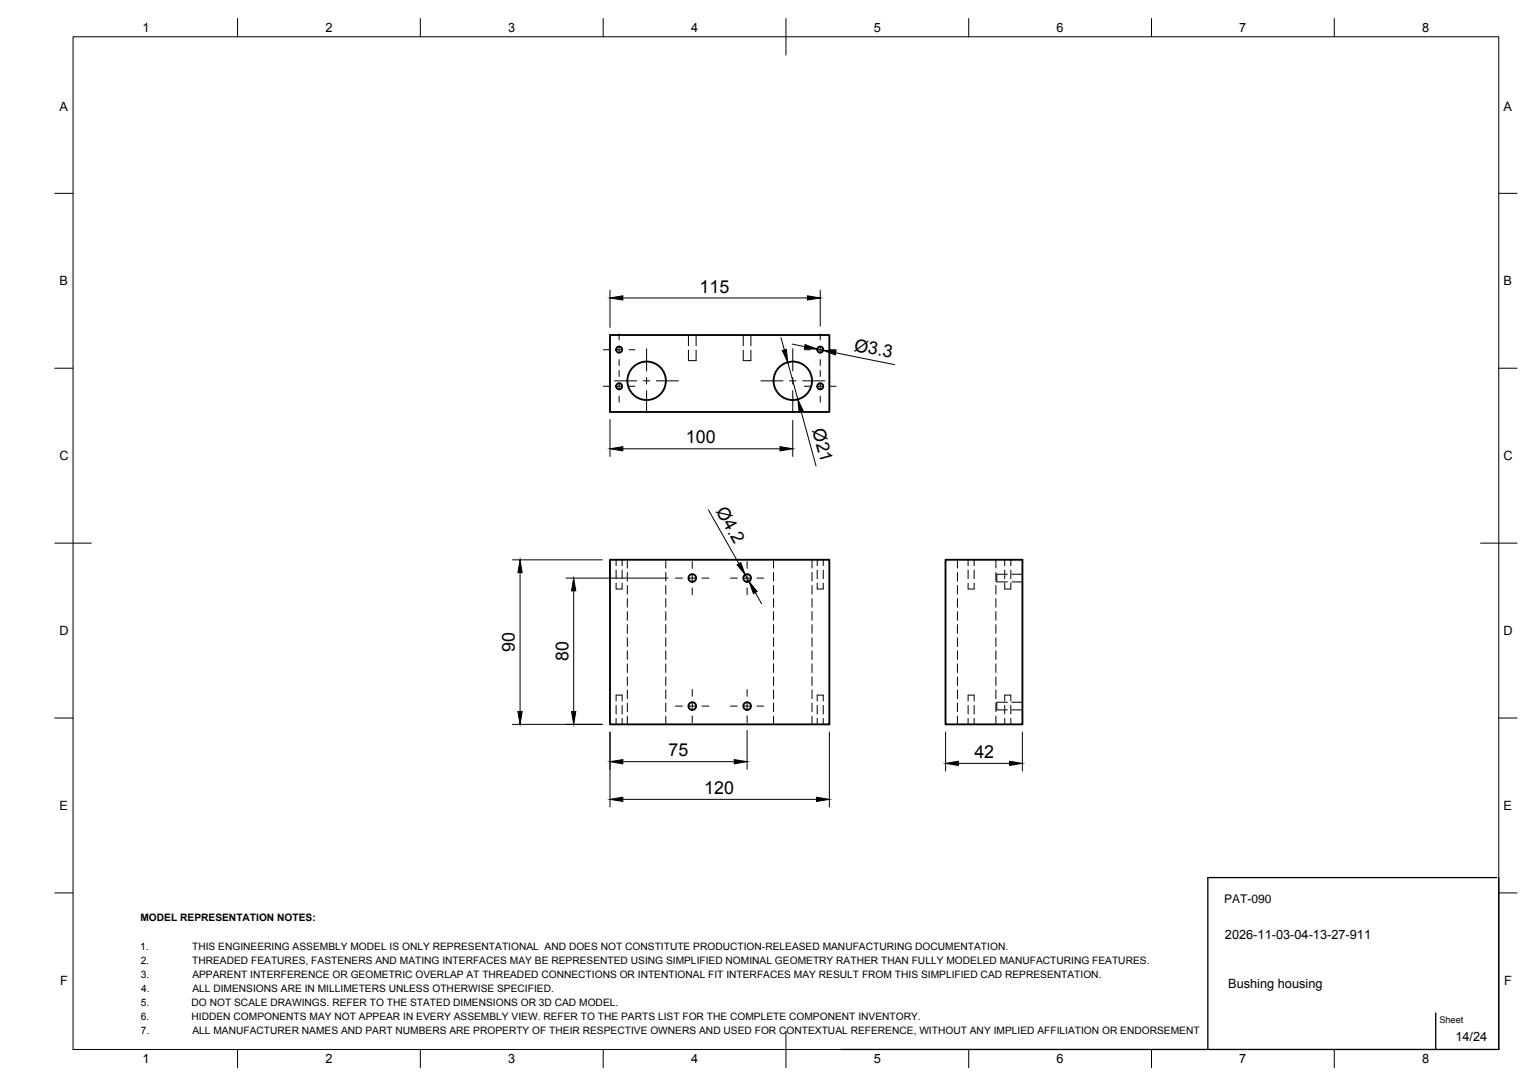
ISO-10303-21;
HEADER;
/* Generated by software containing ST-Developer
 * from STEP Tools, Inc. (www.steptools.com) 
 */

FILE_DESCRIPTION(
/* description */ ('Round-Shaft Linear Stage with Ball Bushings'),
/* implementation_level */ '2;1');

FILE_NAME(
/* name */ 'Bushing housing.step',
/* time_stamp */ '2026-10-27T10:47:55-07:00',
/* author */ (''),
/* organization */ (''),
/* preprocessor_version */ 'ST-DEVELOPER v20.2',
/* originating_system */ 'Autodesk Translation Framework v15.17.0.0',
/* authorisation */ '');

FILE_SCHEMA (('AUTOMOTIVE_DESIGN { 1 0 10303 214 3 1 1 }'));
ENDSEC;

DATA;
#10=MECHANICAL_DESIGN_GEOMETRIC_PRESENTATION_REPRESENTATION('',(#310),#7835);
#268=SHAPE_REPRESENTATION_RELATIONSHIP('SRR','None',#7957,#289);
#289=ADVANCED_BREP_SHAPE_REPRESENTATION('',(#330),#7821);
#310=STYLED_ITEM('',(#8123),#330);
#330=MANIFOLD_SOLID_BREP('Body1',#4401);
#387=FACE_BOUND('',#1046,.T.);
#388=FACE_BOUND('',#1047,.T.);
#389=FACE_BOUND('',#1048,.T.);
#390=FACE_BOUND('',#1049,.T.);
#391=FACE_BOUND('',#1050,.T.);
#392=FACE_BOUND('',#1051,.T.);
#393=FACE_BOUND('',#1054,.T.);
#394=FACE_BOUND('',#1055,.T.);
#395=FACE_BOUND('',#1056,.T.);
#396=FACE_BOUND('',#1057,.T.);
#397=FACE_BOUND('',#1058,.T.);
#398=FACE_BOUND('',#1059,.T.);
#399=FACE_BOUND('',#1061,.T.);
#400=FACE_BOUND('',#1062,.T.);
#401=FACE_BOUND('',#1063,.T.);
#402=FACE_BOUND('',#1064,.T.);
#522=PLANE('',#4827);
#523=PLANE('',#4831);
#524=PLANE('',#4835);
#525=PLANE('',#4839);
#526=PLANE('',#4843);
#527=PLANE('',#4847);
#528=PLANE('',#4851);
#529=PLANE('',#4855);
#530=PLANE('',#4859);
#531=PLANE('',#4863);
#532=PLANE('',#4867);
#533=PLANE('',#4871);
#534=PLANE('',#4878);
#535=PLANE('',#4879);
#536=PLANE('',#4880);
#537=PLANE('',#4881);
#538=PLANE('',#4882);
#539=PLANE('',#4883);
#714=FACE_OUTER_BOUND('',#1018,.T.);
#715=FACE_OUTER_BOUND('',#1019,.T.);
#716=FACE_OUTER_BOUND('',#1020,.T.);
#717=FACE_OUTER_BOUND('',#1021,.T.);
#718=FACE_OUTER_BOUND('',#1022,.T.);
#719=FACE_OUTER_BOUND('',#1023,.T.);
#720=FACE_OUTER_BOUND('',#1024,.T.);
#721=FACE_OUTER_BOUND('',#1025,.T.);
#722=FACE_OUTER_BOUND('',#1026,.T.);
#723=FACE_OUTER_BOUND('',#1027,.T.);
#724=FACE_OUTER_BOUND('',#1028,.T.);
#725=FACE_OUTER_BOUND('',#1029,.T.);
#726=FACE_OUTER_BOUND('',#1030,.T.);
#727=FACE_OUTER_BOUND('',#1031,.T.);
#728=FACE_OUTER_BOUND('',#1032,.T.);
#729=FACE_OUTER_BOUND('',#1033,.T.);
#730=FACE_OUTER_BOUND('',#1034,.T.);
#731=FACE_OUTER_BOUND('',#1035,.T.);
#732=FACE_OUTER_BOUND('',#1036,.T.);
#733=FACE_OUTER_BOUND('',#1037,.T.);
#734=FACE_OUTER_BOUND('',#1038,.T.);
#735=FACE_OUTER_BOUND('',#1039,.T.);
#736=FACE_OUTER_BOUND('',#1040,.T.);
#737=FACE_OUTER_BOUND('',#1041,.T.);
#738=FACE_OUTER_BOUND('',#1042,.T.);
#739=FACE_OUTER_BOUND('',#1043,.T.);
#740=FACE_OUTER_BOUND('',#1044,.T.);
#741=FACE_OUTER_BOUND('',#1045,.T.);
#742=FACE_OUTER_BOUND('',#1052,.T.);
#743=FACE_OUTER_BOUND('',#1053,.T.);
#744=FACE_OUTER_BOUND('',#1060,.T.);
#745=FACE_OUTER_BOUND('',#1065,.T.);
#1018=EDGE_LOOP('',(#3434,#3435,#3436,#3437));
#1019=EDGE_LOOP('',(#3438));
#1020=EDGE_LOOP('',(#3439,#3440,#3441,#3442));
#1021=EDGE_LOOP('',(#3443));
#1022=EDGE_LOOP('',(#3444,#3445,#3446,#3447));
#1023=EDGE_LOOP('',(#3448));
#1024=EDGE_LOOP('',(#3449,#3450,#3451,#3452));
#1025=EDGE_LOOP('',(#3453));
#1026=EDGE_LOOP('',(#3454,#3455,#3456,#3457));
#1027=EDGE_LOOP('',(#3458));
#1028=EDGE_LOOP('',(#3459,#3460,#3461,#3462));
#1029=EDGE_LOOP('',(#3463));
#1030=EDGE_LOOP('',(#3464,#3465,#3466,#3467));
#1031=EDGE_LOOP('',(#3468));
#1032=EDGE_LOOP('',(#3469,#3470,#3471,#3472));
#1033=EDGE_LOOP('',(#3473));
#1034=EDGE_LOOP('',(#3474,#3475,#3476,#3477));
#1035=EDGE_LOOP('',(#3478));
#1036=EDGE_LOOP('',(#3479,#3480,#3481,#3482));
#1037=EDGE_LOOP('',(#3483));
#1038=EDGE_LOOP('',(#3484,#3485,#3486,#3487));
#1039=EDGE_LOOP('',(#3488));
#1040=EDGE_LOOP('',(#3489,#3490,#3491,#3492));
#1041=EDGE_LOOP('',(#3493));
#1042=EDGE_LOOP('',(#3494,#3495,#3496,#3497));
#1043=EDGE_LOOP('',(#3498,#3499,#3500,#3501));
#1044=EDGE_LOOP('',(#3502,#3503,#3504,#3505));
#1045=EDGE_LOOP('',(#3506,#3507,#3508,#3509));
#1046=EDGE_LOOP('',(#3510));
#1047=EDGE_LOOP('',(#3511));
#1048=EDGE_LOOP('',(#3512));
#1049=EDGE_LOOP('',(#3513));
#1050=EDGE_LOOP('',(#3514));
#1051=EDGE_LOOP('',(#3515));
#1052=EDGE_LOOP('',(#3516,#3517,#3518,#3519));
#1053=EDGE_LOOP('',(#3520,#3521,#3522,#3523));
#1054=EDGE_LOOP('',(#3524));
#1055=EDGE_LOOP('',(#3525));
#1056=EDGE_LOOP('',(#3526));
#1057=EDGE_LOOP('',(#3527));
#1058=EDGE_LOOP('',(#3528));
#1059=EDGE_LOOP('',(#3529));
#1060=EDGE_LOOP('',(#3530,#3531,#3532,#3533));
#1061=EDGE_LOOP('',(#3534));
#1062=EDGE_LOOP('',(#3535));
#1063=EDGE_LOOP('',(#3536));
#1064=EDGE_LOOP('',(#3537));
#1065=EDGE_LOOP('',(#3538,#3539,#3540,#3541));
#1404=LINE('',#7049,#1744);
#1405=LINE('',#7056,#1745);
#1406=LINE('',#7063,#1746);
#1407=LINE('',#7070,#1747);
#1408=LINE('',#7077,#1748);
#1409=LINE('',#7084,#1749);
#1410=LINE('',#7091,#1750);
#1411=LINE('',#7098,#1751);
#1412=LINE('',#7105,#1752);
#1413=LINE('',#7112,#1753);
#1414=LINE('',#7119,#1754);
#1415=LINE('',#7126,#1755);
#1416=LINE('',#7133,#1756);
#1417=LINE('',#7139,#1757);
#1418=LINE('',#7144,#1758);
#1419=LINE('',#7146,#1759);
#1420=LINE('',#7148,#1760);
#1421=LINE('',#7149,#1761);
#1422=LINE('',#7152,#1762);
#1423=LINE('',#7154,#1763);
#1424=LINE('',#7155,#1764);
#1425=LINE('',#7158,#1765);
#1426=LINE('',#7160,#1766);
#1427=LINE('',#7161,#1767);
#1428=LINE('',#7163,#1768);
#1429=LINE('',#7164,#1769);
#1744=VECTOR('',#5685,0.165);
#1745=VECTOR('',#5694,0.165);
#1746=VECTOR('',#5703,0.165);
#1747=VECTOR('',#5712,0.165);
#1748=VECTOR('',#5721,0.165);
#1749=VECTOR('',#5730,0.165);
#1750=VECTOR('',#5739,0.165);
#1751=VECTOR('',#5748,0.165);
#1752=VECTOR('',#5757,0.210000000000001);
#1753=VECTOR('',#5766,0.210000000000001);
#1754=VECTOR('',#5775,0.210000000000001);
#1755=VECTOR('',#5784,0.210000000000001);
#1756=VECTOR('',#5793,1.05);
#1757=VECTOR('',#5800,1.05);
#1758=VECTOR('',#5805,1.);
#1759=VECTOR('',#5806,1.);
#1760=VECTOR('',#5807,1.);
#1761=VECTOR('',#5808,1.);
#1762=VECTOR('',#5811,1.);
#1763=VECTOR('',#5812,1.);
#1764=VECTOR('',#5813,1.);
#1765=VECTOR('',#5816,1.);
#1766=VECTOR('',#5817,1.);
#1767=VECTOR('',#5818,1.);
#1768=VECTOR('',#5821,1.);
#1769=VECTOR('',#5822,1.);
#1994=CIRCLE('',#4825,0.165);
#1995=CIRCLE('',#4826,0.165);
#1996=CIRCLE('',#4829,0.165);
#1997=CIRCLE('',#4830,0.165);
#1998=CIRCLE('',#4833,0.165);
#1999=CIRCLE('',#4834,0.165);
#2000=CIRCLE('',#4837,0.165);
#2001=CIRCLE('',#4838,0.165);
#2002=CIRCLE('',#4841,0.165);
#2003=CIRCLE('',#4842,0.165);
#2004=CIRCLE('',#4845,0.165);
#2005=CIRCLE('',#4846,0.165);
#2006=CIRCLE('',#4849,0.165);
#2007=CIRCLE('',#4850,0.165);
#2008=CIRCLE('',#4853,0.165);
#2009=CIRCLE('',#4854,0.165);
#2010=CIRCLE('',#4857,0.210000000000001);
#2011=CIRCLE('',#4858,0.210000000000001);
#2012=CIRCLE('',#4861,0.210000000000001);
#2013=CIRCLE('',#4862,0.210000000000001);
#2014=CIRCLE('',#4865,0.210000000000001);
#2015=CIRCLE('',#4866,0.210000000000001);
#2016=CIRCLE('',#4869,0.210000000000001);
#2017=CIRCLE('',#4870,0.210000000000001);
#2018=CIRCLE('',#4873,1.05);
#2019=CIRCLE('',#4874,1.05);
#2020=CIRCLE('',#4876,1.05);
#2021=CIRCLE('',#4877,1.05);
#2263=VERTEX_POINT('',#7046);
#2264=VERTEX_POINT('',#7048);
#2265=VERTEX_POINT('',#7053);
#2266=VERTEX_POINT('',#7055);
#2267=VERTEX_POINT('',#7060);
#2268=VERTEX_POINT('',#7062);
#2269=VERTEX_POINT('',#7067);
#2270=VERTEX_POINT('',#7069);
#2271=VERTEX_POINT('',#7074);
#2272=VERTEX_POINT('',#7076);
#2273=VERTEX_POINT('',#7081);
#2274=VERTEX_POINT('',#7083);
#2275=VERTEX_POINT('',#7088);
#2276=VERTEX_POINT('',#7090);
#2277=VERTEX_POINT('',#7095);
#2278=VERTEX_POINT('',#7097);
#2279=VERTEX_POINT('',#7102);
#2280=VERTEX_POINT('',#7104);
#2281=VERTEX_POINT('',#7109);
#2282=VERTEX_POINT('',#7111);
#2283=VERTEX_POINT('',#7116);
#2284=VERTEX_POINT('',#7118);
#2285=VERTEX_POINT('',#7123);
#2286=VERTEX_POINT('',#7125);
#2287=VERTEX_POINT('',#7130);
#2288=VERTEX_POINT('',#7132);
#2289=VERTEX_POINT('',#7136);
#2290=VERTEX_POINT('',#7138);
#2291=VERTEX_POINT('',#7142);
#2292=VERTEX_POINT('',#7143);
#2293=VERTEX_POINT('',#7145);
#2294=VERTEX_POINT('',#7147);
#2295=VERTEX_POINT('',#7151);
#2296=VERTEX_POINT('',#7153);
#2297=VERTEX_POINT('',#7157);
#2298=VERTEX_POINT('',#7159);
#2685=EDGE_CURVE('',#2263,#2263,#1994,.T.);
#2686=EDGE_CURVE('',#2263,#2264,#1404,.T.);
#2687=EDGE_CURVE('',#2264,#2264,#1995,.T.);
#2688=EDGE_CURVE('',#2265,#2265,#1996,.T.);
#2689=EDGE_CURVE('',#2265,#2266,#1405,.T.);
#2690=EDGE_CURVE('',#2266,#2266,#1997,.T.);
#2691=EDGE_CURVE('',#2267,#2267,#1998,.T.);
#2692=EDGE_CURVE('',#2267,#2268,#1406,.T.);
#2693=EDGE_CURVE('',#2268,#2268,#1999,.T.);
#2694=EDGE_CURVE('',#2269,#2269,#2000,.T.);
#2695=EDGE_CURVE('',#2269,#2270,#1407,.T.);
#2696=EDGE_CURVE('',#2270,#2270,#2001,.T.);
#2697=EDGE_CURVE('',#2271,#2271,#2002,.T.);
#2698=EDGE_CURVE('',#2271,#2272,#1408,.T.);
#2699=EDGE_CURVE('',#2272,#2272,#2003,.T.);
#2700=EDGE_CURVE('',#2273,#2273,#2004,.T.);
#2701=EDGE_CURVE('',#2273,#2274,#1409,.T.);
#2702=EDGE_CURVE('',#2274,#2274,#2005,.T.);
#2703=EDGE_CURVE('',#2275,#2275,#2006,.T.);
#2704=EDGE_CURVE('',#2275,#2276,#1410,.T.);
#2705=EDGE_CURVE('',#2276,#2276,#2007,.T.);
#2706=EDGE_CURVE('',#2277,#2277,#2008,.T.);
#2707=EDGE_CURVE('',#2277,#2278,#1411,.T.);
#2708=EDGE_CURVE('',#2278,#2278,#2009,.T.);
#2709=EDGE_CURVE('',#2279,#2279,#2010,.T.);
#2710=EDGE_CURVE('',#2279,#2280,#1412,.T.);
#2711=EDGE_CURVE('',#2280,#2280,#2011,.T.);
#2712=EDGE_CURVE('',#2281,#2281,#2012,.T.);
#2713=EDGE_CURVE('',#2281,#2282,#1413,.T.);
#2714=EDGE_CURVE('',#2282,#2282,#2013,.T.);
#2715=EDGE_CURVE('',#2283,#2283,#2014,.T.);
#2716=EDGE_CURVE('',#2283,#2284,#1414,.T.);
#2717=EDGE_CURVE('',#2284,#2284,#2015,.T.);
#2718=EDGE_CURVE('',#2285,#2285,#2016,.T.);
#2719=EDGE_CURVE('',#2285,#2286,#1415,.T.);
#2720=EDGE_CURVE('',#2286,#2286,#2017,.T.);
#2721=EDGE_CURVE('',#2287,#2287,#2018,.T.);
#2722=EDGE_CURVE('',#2287,#2288,#1416,.T.);
#2723=EDGE_CURVE('',#2288,#2288,#2019,.T.);
#2724=EDGE_CURVE('',#2289,#2289,#2020,.T.);
#2725=EDGE_CURVE('',#2289,#2290,#1417,.T.);
#2726=EDGE_CURVE('',#2290,#2290,#2021,.T.);
#2727=EDGE_CURVE('',#2291,#2292,#1418,.T.);
#2728=EDGE_CURVE('',#2292,#2293,#1419,.T.);
#2729=EDGE_CURVE('',#2294,#2293,#1420,.T.);
#2730=EDGE_CURVE('',#2291,#2294,#1421,.T.);
#2731=EDGE_CURVE('',#2295,#2291,#1422,.T.);
#2732=EDGE_CURVE('',#2296,#2294,#1423,.T.);
#2733=EDGE_CURVE('',#2295,#2296,#1424,.T.);
#2734=EDGE_CURVE('',#2297,#2295,#1425,.T.);
#2735=EDGE_CURVE('',#2298,#2296,#1426,.T.);
#2736=EDGE_CURVE('',#2297,#2298,#1427,.T.);
#2737=EDGE_CURVE('',#2292,#2297,#1428,.T.);
#2738=EDGE_CURVE('',#2293,#2298,#1429,.T.);
#3434=ORIENTED_EDGE('',*,*,#2685,.F.);
#3435=ORIENTED_EDGE('',*,*,#2686,.T.);
#3436=ORIENTED_EDGE('',*,*,#2687,.F.);
#3437=ORIENTED_EDGE('',*,*,#2686,.F.);
#3438=ORIENTED_EDGE('',*,*,#2685,.T.);
#3439=ORIENTED_EDGE('',*,*,#2688,.F.);
#3440=ORIENTED_EDGE('',*,*,#2689,.T.);
#3441=ORIENTED_EDGE('',*,*,#2690,.F.);
#3442=ORIENTED_EDGE('',*,*,#2689,.F.);
#3443=ORIENTED_EDGE('',*,*,#2688,.T.);
#3444=ORIENTED_EDGE('',*,*,#2691,.F.);
#3445=ORIENTED_EDGE('',*,*,#2692,.T.);
#3446=ORIENTED_EDGE('',*,*,#2693,.F.);
#3447=ORIENTED_EDGE('',*,*,#2692,.F.);
#3448=ORIENTED_EDGE('',*,*,#2691,.T.);
#3449=ORIENTED_EDGE('',*,*,#2694,.F.);
#3450=ORIENTED_EDGE('',*,*,#2695,.T.);
#3451=ORIENTED_EDGE('',*,*,#2696,.F.);
#3452=ORIENTED_EDGE('',*,*,#2695,.F.);
#3453=ORIENTED_EDGE('',*,*,#2694,.T.);
#3454=ORIENTED_EDGE('',*,*,#2697,.F.);
#3455=ORIENTED_EDGE('',*,*,#2698,.T.);
#3456=ORIENTED_EDGE('',*,*,#2699,.T.);
#3457=ORIENTED_EDGE('',*,*,#2698,.F.);
#3458=ORIENTED_EDGE('',*,*,#2699,.F.);
#3459=ORIENTED_EDGE('',*,*,#2700,.F.);
#3460=ORIENTED_EDGE('',*,*,#2701,.T.);
#3461=ORIENTED_EDGE('',*,*,#2702,.T.);
#3462=ORIENTED_EDGE('',*,*,#2701,.F.);
#3463=ORIENTED_EDGE('',*,*,#2702,.F.);
#3464=ORIENTED_EDGE('',*,*,#2703,.F.);
#3465=ORIENTED_EDGE('',*,*,#2704,.T.);
#3466=ORIENTED_EDGE('',*,*,#2705,.T.);
#3467=ORIENTED_EDGE('',*,*,#2704,.F.);
#3468=ORIENTED_EDGE('',*,*,#2705,.F.);
#3469=ORIENTED_EDGE('',*,*,#2706,.F.);
#3470=ORIENTED_EDGE('',*,*,#2707,.T.);
#3471=ORIENTED_EDGE('',*,*,#2708,.T.);
#3472=ORIENTED_EDGE('',*,*,#2707,.F.);
#3473=ORIENTED_EDGE('',*,*,#2708,.F.);
#3474=ORIENTED_EDGE('',*,*,#2709,.F.);
#3475=ORIENTED_EDGE('',*,*,#2710,.T.);
#3476=ORIENTED_EDGE('',*,*,#2711,.F.);
#3477=ORIENTED_EDGE('',*,*,#2710,.F.);
#3478=ORIENTED_EDGE('',*,*,#2709,.T.);
#3479=ORIENTED_EDGE('',*,*,#2712,.F.);
#3480=ORIENTED_EDGE('',*,*,#2713,.T.);
#3481=ORIENTED_EDGE('',*,*,#2714,.F.);
#3482=ORIENTED_EDGE('',*,*,#2713,.F.);
#3483=ORIENTED_EDGE('',*,*,#2712,.T.);
#3484=ORIENTED_EDGE('',*,*,#2715,.F.);
#3485=ORIENTED_EDGE('',*,*,#2716,.T.);
#3486=ORIENTED_EDGE('',*,*,#2717,.F.);
#3487=ORIENTED_EDGE('',*,*,#2716,.F.);
#3488=ORIENTED_EDGE('',*,*,#2715,.T.);
#3489=ORIENTED_EDGE('',*,*,#2718,.F.);
#3490=ORIENTED_EDGE('',*,*,#2719,.T.);
#3491=ORIENTED_EDGE('',*,*,#2720,.F.);
#3492=ORIENTED_EDGE('',*,*,#2719,.F.);
#3493=ORIENTED_EDGE('',*,*,#2718,.T.);
#3494=ORIENTED_EDGE('',*,*,#2721,.F.);
#3495=ORIENTED_EDGE('',*,*,#2722,.T.);
#3496=ORIENTED_EDGE('',*,*,#2723,.F.);
#3497=ORIENTED_EDGE('',*,*,#2722,.F.);
#3498=ORIENTED_EDGE('',*,*,#2724,.F.);
#3499=ORIENTED_EDGE('',*,*,#2725,.T.);
#3500=ORIENTED_EDGE('',*,*,#2726,.F.);
#3501=ORIENTED_EDGE('',*,*,#2725,.F.);
#3502=ORIENTED_EDGE('',*,*,#2727,.T.);
#3503=ORIENTED_EDGE('',*,*,#2728,.T.);
#3504=ORIENTED_EDGE('',*,*,#2729,.F.);
#3505=ORIENTED_EDGE('',*,*,#2730,.F.);
#3506=ORIENTED_EDGE('',*,*,#2731,.T.);
#3507=ORIENTED_EDGE('',*,*,#2730,.T.);
#3508=ORIENTED_EDGE('',*,*,#2732,.F.);
#3509=ORIENTED_EDGE('',*,*,#2733,.F.);
#3510=ORIENTED_EDGE('',*,*,#2726,.T.);
#3511=ORIENTED_EDGE('',*,*,#2723,.T.);
#3512=ORIENTED_EDGE('',*,*,#2696,.T.);
#3513=ORIENTED_EDGE('',*,*,#2693,.T.);
#3514=ORIENTED_EDGE('',*,*,#2690,.T.);
#3515=ORIENTED_EDGE('',*,*,#2687,.T.);
#3516=ORIENTED_EDGE('',*,*,#2734,.T.);
#3517=ORIENTED_EDGE('',*,*,#2733,.T.);
#3518=ORIENTED_EDGE('',*,*,#2735,.F.);
#3519=ORIENTED_EDGE('',*,*,#2736,.F.);
#3520=ORIENTED_EDGE('',*,*,#2737,.T.);
#3521=ORIENTED_EDGE('',*,*,#2736,.T.);
#3522=ORIENTED_EDGE('',*,*,#2738,.F.);
#3523=ORIENTED_EDGE('',*,*,#2728,.F.);
#3524=ORIENTED_EDGE('',*,*,#2724,.T.);
#3525=ORIENTED_EDGE('',*,*,#2721,.T.);
#3526=ORIENTED_EDGE('',*,*,#2706,.T.);
#3527=ORIENTED_EDGE('',*,*,#2703,.T.);
#3528=ORIENTED_EDGE('',*,*,#2700,.T.);
#3529=ORIENTED_EDGE('',*,*,#2697,.T.);
#3530=ORIENTED_EDGE('',*,*,#2738,.T.);
#3531=ORIENTED_EDGE('',*,*,#2735,.T.);
#3532=ORIENTED_EDGE('',*,*,#2732,.T.);
#3533=ORIENTED_EDGE('',*,*,#2729,.T.);
#3534=ORIENTED_EDGE('',*,*,#2711,.T.);
#3535=ORIENTED_EDGE('',*,*,#2714,.T.);
#3536=ORIENTED_EDGE('',*,*,#2717,.T.);
#3537=ORIENTED_EDGE('',*,*,#2720,.T.);
#3538=ORIENTED_EDGE('',*,*,#2737,.F.);
#3539=ORIENTED_EDGE('',*,*,#2727,.F.);
#3540=ORIENTED_EDGE('',*,*,#2731,.F.);
#3541=ORIENTED_EDGE('',*,*,#2734,.F.);
#4082=CYLINDRICAL_SURFACE('',#4824,0.165);
#4083=CYLINDRICAL_SURFACE('',#4828,0.165);
#4084=CYLINDRICAL_SURFACE('',#4832,0.165);
#4085=CYLINDRICAL_SURFACE('',#4836,0.165);
#4086=CYLINDRICAL_SURFACE('',#4840,0.165);
#4087=CYLINDRICAL_SURFACE('',#4844,0.165);
#4088=CYLINDRICAL_SURFACE('',#4848,0.165);
#4089=CYLINDRICAL_SURFACE('',#4852,0.165);
#4090=CYLINDRICAL_SURFACE('',#4856,0.210000000000001);
#4091=CYLINDRICAL_SURFACE('',#4860,0.210000000000001);
#4092=CYLINDRICAL_SURFACE('',#4864,0.210000000000001);
#4093=CYLINDRICAL_SURFACE('',#4868,0.210000000000001);
#4094=CYLINDRICAL_SURFACE('',#4872,1.05);
#4095=CYLINDRICAL_SURFACE('',#4875,1.05);
#4233=ADVANCED_FACE('',(#714),#4082,.F.);
#4234=ADVANCED_FACE('',(#715),#522,.T.);
#4235=ADVANCED_FACE('',(#716),#4083,.F.);
#4236=ADVANCED_FACE('',(#717),#523,.T.);
#4237=ADVANCED_FACE('',(#718),#4084,.F.);
#4238=ADVANCED_FACE('',(#719),#524,.T.);
#4239=ADVANCED_FACE('',(#720),#4085,.F.);
#4240=ADVANCED_FACE('',(#721),#525,.T.);
#4241=ADVANCED_FACE('',(#722),#4086,.F.);
#4242=ADVANCED_FACE('',(#723),#526,.F.);
#4243=ADVANCED_FACE('',(#724),#4087,.F.);
#4244=ADVANCED_FACE('',(#725),#527,.F.);
#4245=ADVANCED_FACE('',(#726),#4088,.F.);
#4246=ADVANCED_FACE('',(#727),#528,.F.);
#4247=ADVANCED_FACE('',(#728),#4089,.F.);
#4248=ADVANCED_FACE('',(#729),#529,.F.);
#4249=ADVANCED_FACE('',(#730),#4090,.F.);
#4250=ADVANCED_FACE('',(#731),#530,.T.);
#4251=ADVANCED_FACE('',(#732),#4091,.F.);
#4252=ADVANCED_FACE('',(#733),#531,.T.);
#4253=ADVANCED_FACE('',(#734),#4092,.F.);
#4254=ADVANCED_FACE('',(#735),#532,.T.);
#4255=ADVANCED_FACE('',(#736),#4093,.F.);
#4256=ADVANCED_FACE('',(#737),#533,.T.);
#4257=ADVANCED_FACE('',(#738),#4094,.F.);
#4258=ADVANCED_FACE('',(#739),#4095,.F.);
#4259=ADVANCED_FACE('',(#740),#534,.T.);
#4260=ADVANCED_FACE('',(#741,#387,#388,#389,#390,#391,#392),#535,.T.);
#4261=ADVANCED_FACE('',(#742),#536,.T.);
#4262=ADVANCED_FACE('',(#743,#393,#394,#395,#396,#397,#398),#537,.T.);
#4263=ADVANCED_FACE('',(#744,#399,#400,#401,#402),#538,.T.);
#4264=ADVANCED_FACE('',(#745),#539,.F.);
#4401=CLOSED_SHELL('',(#4233,#4234,#4235,#4236,#4237,#4238,#4239,#4240,
#4241,#4242,#4243,#4244,#4245,#4246,#4247,#4248,#4249,#4250,#4251,#4252,
#4253,#4254,#4255,#4256,#4257,#4258,#4259,#4260,#4261,#4262,#4263,#4264));
#4823=AXIS2_PLACEMENT_3D('',#7044,#5679,#5680);
#4824=AXIS2_PLACEMENT_3D('',#7045,#5681,#5682);
#4825=AXIS2_PLACEMENT_3D('',#7047,#5683,#5684);
#4826=AXIS2_PLACEMENT_3D('',#7050,#5686,#5687);
#4827=AXIS2_PLACEMENT_3D('',#7051,#5688,#5689);
#4828=AXIS2_PLACEMENT_3D('',#7052,#5690,#5691);
#4829=AXIS2_PLACEMENT_3D('',#7054,#5692,#5693);
#4830=AXIS2_PLACEMENT_3D('',#7057,#5695,#5696);
#4831=AXIS2_PLACEMENT_3D('',#7058,#5697,#5698);
#4832=AXIS2_PLACEMENT_3D('',#7059,#5699,#5700);
#4833=AXIS2_PLACEMENT_3D('',#7061,#5701,#5702);
#4834=AXIS2_PLACEMENT_3D('',#7064,#5704,#5705);
#4835=AXIS2_PLACEMENT_3D('',#7065,#5706,#5707);
#4836=AXIS2_PLACEMENT_3D('',#7066,#5708,#5709);
#4837=AXIS2_PLACEMENT_3D('',#7068,#5710,#5711);
#4838=AXIS2_PLACEMENT_3D('',#7071,#5713,#5714);
#4839=AXIS2_PLACEMENT_3D('',#7072,#5715,#5716);
#4840=AXIS2_PLACEMENT_3D('',#7073,#5717,#5718);
#4841=AXIS2_PLACEMENT_3D('',#7075,#5719,#5720);
#4842=AXIS2_PLACEMENT_3D('',#7078,#5722,#5723);
#4843=AXIS2_PLACEMENT_3D('',#7079,#5724,#5725);
#4844=AXIS2_PLACEMENT_3D('',#7080,#5726,#5727);
#4845=AXIS2_PLACEMENT_3D('',#7082,#5728,#5729);
#4846=AXIS2_PLACEMENT_3D('',#7085,#5731,#5732);
#4847=AXIS2_PLACEMENT_3D('',#7086,#5733,#5734);
#4848=AXIS2_PLACEMENT_3D('',#7087,#5735,#5736);
#4849=AXIS2_PLACEMENT_3D('',#7089,#5737,#5738);
#4850=AXIS2_PLACEMENT_3D('',#7092,#5740,#5741);
#4851=AXIS2_PLACEMENT_3D('',#7093,#5742,#5743);
#4852=AXIS2_PLACEMENT_3D('',#7094,#5744,#5745);
#4853=AXIS2_PLACEMENT_3D('',#7096,#5746,#5747);
#4854=AXIS2_PLACEMENT_3D('',#7099,#5749,#5750);
#4855=AXIS2_PLACEMENT_3D('',#7100,#5751,#5752);
#4856=AXIS2_PLACEMENT_3D('',#7101,#5753,#5754);
#4857=AXIS2_PLACEMENT_3D('',#7103,#5755,#5756);
#4858=AXIS2_PLACEMENT_3D('',#7106,#5758,#5759);
#4859=AXIS2_PLACEMENT_3D('',#7107,#5760,#5761);
#4860=AXIS2_PLACEMENT_3D('',#7108,#5762,#5763);
#4861=AXIS2_PLACEMENT_3D('',#7110,#5764,#5765);
#4862=AXIS2_PLACEMENT_3D('',#7113,#5767,#5768);
#4863=AXIS2_PLACEMENT_3D('',#7114,#5769,#5770);
#4864=AXIS2_PLACEMENT_3D('',#7115,#5771,#5772);
#4865=AXIS2_PLACEMENT_3D('',#7117,#5773,#5774);
#4866=AXIS2_PLACEMENT_3D('',#7120,#5776,#5777);
#4867=AXIS2_PLACEMENT_3D('',#7121,#5778,#5779);
#4868=AXIS2_PLACEMENT_3D('',#7122,#5780,#5781);
#4869=AXIS2_PLACEMENT_3D('',#7124,#5782,#5783);
#4870=AXIS2_PLACEMENT_3D('',#7127,#5785,#5786);
#4871=AXIS2_PLACEMENT_3D('',#7128,#5787,#5788);
#4872=AXIS2_PLACEMENT_3D('',#7129,#5789,#5790);
#4873=AXIS2_PLACEMENT_3D('',#7131,#5791,#5792);
#4874=AXIS2_PLACEMENT_3D('',#7134,#5794,#5795);
#4875=AXIS2_PLACEMENT_3D('',#7135,#5796,#5797);
#4876=AXIS2_PLACEMENT_3D('',#7137,#5798,#5799);
#4877=AXIS2_PLACEMENT_3D('',#7140,#5801,#5802);
#4878=AXIS2_PLACEMENT_3D('',#7141,#5803,#5804);
#4879=AXIS2_PLACEMENT_3D('',#7150,#5809,#5810);
#4880=AXIS2_PLACEMENT_3D('',#7156,#5814,#5815);
#4881=AXIS2_PLACEMENT_3D('',#7162,#5819,#5820);
#4882=AXIS2_PLACEMENT_3D('',#7165,#5823,#5824);
#4883=AXIS2_PLACEMENT_3D('',#7166,#5825,#5826);
#5679=DIRECTION('axis',(0.,0.,1.));
#5680=DIRECTION('refdir',(1.,0.,0.));
#5681=DIRECTION('center_axis',(1.,0.,0.));
#5682=DIRECTION('ref_axis',(0.,0.,-1.));
#5683=DIRECTION('center_axis',(1.,0.,0.));
#5684=DIRECTION('ref_axis',(0.,0.,-1.));
#5685=DIRECTION('',(1.,0.,0.));
#5686=DIRECTION('center_axis',(-1.,0.,0.));
#5687=DIRECTION('ref_axis',(0.,0.,-1.));
#5688=DIRECTION('center_axis',(1.,0.,0.));
#5689=DIRECTION('ref_axis',(0.,0.,-1.));
#5690=DIRECTION('center_axis',(1.,0.,0.));
#5691=DIRECTION('ref_axis',(0.,0.,-1.));
#5692=DIRECTION('center_axis',(1.,0.,0.));
#5693=DIRECTION('ref_axis',(0.,0.,-1.));
#5694=DIRECTION('',(1.,0.,0.));
#5695=DIRECTION('center_axis',(-1.,0.,0.));
#5696=DIRECTION('ref_axis',(0.,0.,-1.));
#5697=DIRECTION('center_axis',(1.,0.,0.));
#5698=DIRECTION('ref_axis',(0.,0.,-1.));
#5699=DIRECTION('center_axis',(1.,0.,0.));
#5700=DIRECTION('ref_axis',(0.,0.,-1.));
#5701=DIRECTION('center_axis',(1.,0.,0.));
#5702=DIRECTION('ref_axis',(0.,0.,-1.));
#5703=DIRECTION('',(1.,0.,0.));
#5704=DIRECTION('center_axis',(-1.,0.,0.));
#5705=DIRECTION('ref_axis',(0.,0.,-1.));
#5706=DIRECTION('center_axis',(1.,0.,0.));
#5707=DIRECTION('ref_axis',(0.,0.,-1.));
#5708=DIRECTION('center_axis',(1.,0.,0.));
#5709=DIRECTION('ref_axis',(0.,0.,-1.));
#5710=DIRECTION('center_axis',(1.,0.,0.));
#5711=DIRECTION('ref_axis',(0.,0.,-1.));
#5712=DIRECTION('',(1.,0.,0.));
#5713=DIRECTION('center_axis',(-1.,0.,0.));
#5714=DIRECTION('ref_axis',(0.,0.,-1.));
#5715=DIRECTION('center_axis',(1.,0.,0.));
#5716=DIRECTION('ref_axis',(0.,0.,-1.));
#5717=DIRECTION('center_axis',(1.,0.,0.));
#5718=DIRECTION('ref_axis',(0.,0.,-1.));
#5719=DIRECTION('center_axis',(1.,0.,0.));
#5720=DIRECTION('ref_axis',(0.,0.,-1.));
#5721=DIRECTION('',(1.,0.,0.));
#5722=DIRECTION('center_axis',(1.,0.,0.));
#5723=DIRECTION('ref_axis',(0.,0.,-1.));
#5724=DIRECTION('center_axis',(1.,0.,0.));
#5725=DIRECTION('ref_axis',(0.,0.,-1.));
#5726=DIRECTION('center_axis',(1.,0.,0.));
#5727=DIRECTION('ref_axis',(0.,0.,-1.));
#5728=DIRECTION('center_axis',(1.,0.,0.));
#5729=DIRECTION('ref_axis',(0.,0.,-1.));
#5730=DIRECTION('',(1.,0.,0.));
#5731=DIRECTION('center_axis',(1.,0.,0.));
#5732=DIRECTION('ref_axis',(0.,0.,-1.));
#5733=DIRECTION('center_axis',(1.,0.,0.));
#5734=DIRECTION('ref_axis',(0.,0.,-1.));
#5735=DIRECTION('center_axis',(1.,0.,0.));
#5736=DIRECTION('ref_axis',(0.,0.,-1.));
#5737=DIRECTION('center_axis',(1.,0.,0.));
#5738=DIRECTION('ref_axis',(0.,0.,-1.));
#5739=DIRECTION('',(1.,0.,0.));
#5740=DIRECTION('center_axis',(1.,0.,0.));
#5741=DIRECTION('ref_axis',(0.,0.,-1.));
#5742=DIRECTION('center_axis',(1.,0.,0.));
#5743=DIRECTION('ref_axis',(0.,0.,-1.));
#5744=DIRECTION('center_axis',(1.,0.,0.));
#5745=DIRECTION('ref_axis',(0.,0.,-1.));
#5746=DIRECTION('center_axis',(1.,0.,0.));
#5747=DIRECTION('ref_axis',(0.,0.,-1.));
#5748=DIRECTION('',(1.,0.,0.));
#5749=DIRECTION('center_axis',(1.,0.,0.));
#5750=DIRECTION('ref_axis',(0.,0.,-1.));
#5751=DIRECTION('center_axis',(1.,0.,0.));
#5752=DIRECTION('ref_axis',(0.,0.,-1.));
#5753=DIRECTION('center_axis',(0.,0.,1.));
#5754=DIRECTION('ref_axis',(1.,0.,0.));
#5755=DIRECTION('center_axis',(0.,0.,1.));
#5756=DIRECTION('ref_axis',(1.,0.,0.));
#5757=DIRECTION('',(0.,0.,1.));
#5758=DIRECTION('center_axis',(0.,0.,-1.));
#5759=DIRECTION('ref_axis',(1.,0.,0.));
#5760=DIRECTION('center_axis',(0.,0.,1.));
#5761=DIRECTION('ref_axis',(1.,0.,0.));
#5762=DIRECTION('center_axis',(0.,0.,1.));
#5763=DIRECTION('ref_axis',(1.,0.,0.));
#5764=DIRECTION('center_axis',(0.,0.,1.));
#5765=DIRECTION('ref_axis',(1.,0.,0.));
#5766=DIRECTION('',(0.,0.,1.));
#5767=DIRECTION('center_axis',(0.,0.,-1.));
#5768=DIRECTION('ref_axis',(1.,0.,0.));
#5769=DIRECTION('center_axis',(0.,0.,1.));
#5770=DIRECTION('ref_axis',(1.,0.,0.));
#5771=DIRECTION('center_axis',(0.,0.,1.));
#5772=DIRECTION('ref_axis',(1.,0.,0.));
#5773=DIRECTION('center_axis',(0.,0.,1.));
#5774=DIRECTION('ref_axis',(1.,0.,0.));
#5775=DIRECTION('',(0.,0.,1.));
#5776=DIRECTION('center_axis',(0.,0.,-1.));
#5777=DIRECTION('ref_axis',(1.,0.,0.));
#5778=DIRECTION('center_axis',(0.,0.,1.));
#5779=DIRECTION('ref_axis',(1.,0.,0.));
#5780=DIRECTION('center_axis',(0.,0.,1.));
#5781=DIRECTION('ref_axis',(1.,0.,0.));
#5782=DIRECTION('center_axis',(0.,0.,1.));
#5783=DIRECTION('ref_axis',(1.,0.,0.));
#5784=DIRECTION('',(0.,0.,1.));
#5785=DIRECTION('center_axis',(0.,0.,-1.));
#5786=DIRECTION('ref_axis',(1.,0.,0.));
#5787=DIRECTION('center_axis',(0.,0.,1.));
#5788=DIRECTION('ref_axis',(1.,0.,0.));
#5789=DIRECTION('center_axis',(1.,0.,0.));
#5790=DIRECTION('ref_axis',(0.,0.,-1.));
#5791=DIRECTION('center_axis',(1.,0.,0.));
#5792=DIRECTION('ref_axis',(0.,0.,-1.));
#5793=DIRECTION('',(1.,0.,0.));
#5794=DIRECTION('center_axis',(-1.,0.,0.));
#5795=DIRECTION('ref_axis',(0.,0.,-1.));
#5796=DIRECTION('center_axis',(1.,0.,0.));
#5797=DIRECTION('ref_axis',(0.,0.,-1.));
#5798=DIRECTION('center_axis',(1.,0.,0.));
#5799=DIRECTION('ref_axis',(0.,0.,-1.));
#5800=DIRECTION('',(1.,0.,0.));
#5801=DIRECTION('center_axis',(-1.,0.,0.));
#5802=DIRECTION('ref_axis',(0.,0.,-1.));
#5803=DIRECTION('center_axis',(0.,1.,0.));
#5804=DIRECTION('ref_axis',(-1.,0.,0.));
#5805=DIRECTION('',(-1.,0.,0.));
#5806=DIRECTION('',(0.,0.,1.));
#5807=DIRECTION('',(-1.,0.,0.));
#5808=DIRECTION('',(0.,0.,1.));
#5809=DIRECTION('center_axis',(1.,0.,0.));
#5810=DIRECTION('ref_axis',(0.,1.,0.));
#5811=DIRECTION('',(0.,1.,0.));
#5812=DIRECTION('',(0.,1.,0.));
#5813=DIRECTION('',(0.,0.,1.));
#5814=DIRECTION('center_axis',(0.,-1.,0.));
#5815=DIRECTION('ref_axis',(1.,0.,0.));
#5816=DIRECTION('',(1.,0.,0.));
#5817=DIRECTION('',(1.,0.,0.));
#5818=DIRECTION('',(0.,0.,1.));
#5819=DIRECTION('center_axis',(-1.,0.,0.));
#5820=DIRECTION('ref_axis',(0.,-1.,0.));
#5821=DIRECTION('',(0.,-1.,0.));
#5822=DIRECTION('',(0.,-1.,0.));
#5823=DIRECTION('center_axis',(0.,0.,1.));
#5824=DIRECTION('ref_axis',(1.,0.,0.));
#5825=DIRECTION('center_axis',(0.,0.,1.));
#5826=DIRECTION('ref_axis',(1.,0.,0.));
#7044=CARTESIAN_POINT('',(0.,0.,0.));
#7045=CARTESIAN_POINT('Origin',(17.9,5.5,3.));
#7046=CARTESIAN_POINT('',(17.9,5.5,3.165));
#7047=CARTESIAN_POINT('Origin',(17.9,5.5,3.));
#7048=CARTESIAN_POINT('',(19.5,5.5,3.165));
#7049=CARTESIAN_POINT('',(17.9,5.5,3.165));
#7050=CARTESIAN_POINT('Origin',(19.5,5.5,3.));
#7051=CARTESIAN_POINT('Origin',(17.9,5.5,3.));
#7052=CARTESIAN_POINT('Origin',(17.9,-5.5,5.));
#7053=CARTESIAN_POINT('',(17.9,-5.5,5.165));
#7054=CARTESIAN_POINT('Origin',(17.9,-5.5,5.));
#7055=CARTESIAN_POINT('',(19.5,-5.5,5.165));
#7056=CARTESIAN_POINT('',(17.9,-5.5,5.165));
#7057=CARTESIAN_POINT('Origin',(19.5,-5.5,5.));
#7058=CARTESIAN_POINT('Origin',(17.9,-5.5,5.));
#7059=CARTESIAN_POINT('Origin',(17.9,-5.5,3.));
#7060=CARTESIAN_POINT('',(17.9,-5.5,3.165));
#7061=CARTESIAN_POINT('Origin',(17.9,-5.5,3.));
#7062=CARTESIAN_POINT('',(19.5,-5.5,3.165));
#7063=CARTESIAN_POINT('',(17.9,-5.5,3.165));
#7064=CARTESIAN_POINT('Origin',(19.5,-5.5,3.));
#7065=CARTESIAN_POINT('Origin',(17.9,-5.5,3.));
#7066=CARTESIAN_POINT('Origin',(17.9,5.5,5.));
#7067=CARTESIAN_POINT('',(17.9,5.5,5.165));
#7068=CARTESIAN_POINT('Origin',(17.9,5.5,5.));
#7069=CARTESIAN_POINT('',(19.5,5.5,5.165));
#7070=CARTESIAN_POINT('',(17.9,5.5,5.165));
#7071=CARTESIAN_POINT('Origin',(19.5,5.5,5.));
#7072=CARTESIAN_POINT('Origin',(17.9,5.5,5.));
#7073=CARTESIAN_POINT('Origin',(10.5,5.5,3.));
#7074=CARTESIAN_POINT('',(10.5,5.5,3.165));
#7075=CARTESIAN_POINT('Origin',(10.5,5.5,3.));
#7076=CARTESIAN_POINT('',(12.1,5.5,3.165));
#7077=CARTESIAN_POINT('',(10.5,5.5,3.165));
#7078=CARTESIAN_POINT('Origin',(12.1,5.5,3.));
#7079=CARTESIAN_POINT('Origin',(12.1,5.5,3.));
#7080=CARTESIAN_POINT('Origin',(10.5,-5.5,5.));
#7081=CARTESIAN_POINT('',(10.5,-5.5,5.165));
#7082=CARTESIAN_POINT('Origin',(10.5,-5.5,5.));
#7083=CARTESIAN_POINT('',(12.1,-5.5,5.165));
#7084=CARTESIAN_POINT('',(10.5,-5.5,5.165));
#7085=CARTESIAN_POINT('Origin',(12.1,-5.5,5.));
#7086=CARTESIAN_POINT('Origin',(12.1,-5.5,5.));
#7087=CARTESIAN_POINT('Origin',(10.5,-5.5,3.));
#7088=CARTESIAN_POINT('',(10.5,-5.5,3.165));
#7089=CARTESIAN_POINT('Origin',(10.5,-5.5,3.));
#7090=CARTESIAN_POINT('',(12.1,-5.5,3.165));
#7091=CARTESIAN_POINT('',(10.5,-5.5,3.165));
#7092=CARTESIAN_POINT('Origin',(12.1,-5.5,3.));
#7093=CARTESIAN_POINT('Origin',(12.1,-5.5,3.));
#7094=CARTESIAN_POINT('Origin',(10.5,5.5,5.));
#7095=CARTESIAN_POINT('',(10.5,5.5,5.165));
#7096=CARTESIAN_POINT('Origin',(10.5,5.5,5.));
#7097=CARTESIAN_POINT('',(12.1,5.5,5.165));
#7098=CARTESIAN_POINT('',(10.5,5.5,5.165));
#7099=CARTESIAN_POINT('Origin',(12.1,5.5,5.));
#7100=CARTESIAN_POINT('Origin',(12.1,5.5,5.));
#7101=CARTESIAN_POINT('Origin',(18.5,-1.5,4.4));
#7102=CARTESIAN_POINT('',(18.29,-1.5,4.4));
#7103=CARTESIAN_POINT('Origin',(18.5,-1.5,4.4));
#7104=CARTESIAN_POINT('',(18.29,-1.5,5.8));
#7105=CARTESIAN_POINT('',(18.29,-1.5,4.4));
#7106=CARTESIAN_POINT('Origin',(18.5,-1.5,5.8));
#7107=CARTESIAN_POINT('Origin',(18.5,-1.5,4.4));
#7108=CARTESIAN_POINT('Origin',(11.5,1.5,4.4));
#7109=CARTESIAN_POINT('',(11.29,1.5,4.4));
#7110=CARTESIAN_POINT('Origin',(11.5,1.5,4.4));
#7111=CARTESIAN_POINT('',(11.29,1.5,5.8));
#7112=CARTESIAN_POINT('',(11.29,1.5,4.4));
#7113=CARTESIAN_POINT('Origin',(11.5,1.5,5.8));
#7114=CARTESIAN_POINT('Origin',(11.5,1.5,4.4));
#7115=CARTESIAN_POINT('Origin',(11.5,-1.5,4.4));
#7116=CARTESIAN_POINT('',(11.29,-1.5,4.4));
#7117=CARTESIAN_POINT('Origin',(11.5,-1.5,4.4));
#7118=CARTESIAN_POINT('',(11.29,-1.5,5.8));
#7119=CARTESIAN_POINT('',(11.29,-1.5,4.4));
#7120=CARTESIAN_POINT('Origin',(11.5,-1.5,5.8));
#7121=CARTESIAN_POINT('Origin',(11.5,-1.5,4.4));
#7122=CARTESIAN_POINT('Origin',(18.5,1.5,4.4));
#7123=CARTESIAN_POINT('',(18.29,1.5,4.4));
#7124=CARTESIAN_POINT('Origin',(18.5,1.5,4.4));
#7125=CARTESIAN_POINT('',(18.29,1.5,5.8));
#7126=CARTESIAN_POINT('',(18.29,1.5,4.4));
#7127=CARTESIAN_POINT('Origin',(18.5,1.5,5.8));
#7128=CARTESIAN_POINT('Origin',(18.5,1.5,4.4));
#7129=CARTESIAN_POINT('Origin',(10.4,-4.,3.3));
#7130=CARTESIAN_POINT('',(10.5,-4.,4.35));
#7131=CARTESIAN_POINT('Origin',(10.5,-4.,3.3));
#7132=CARTESIAN_POINT('',(19.5,-4.,4.35));
#7133=CARTESIAN_POINT('',(10.4,-4.,4.35));
#7134=CARTESIAN_POINT('Origin',(19.5,-4.,3.3));
#7135=CARTESIAN_POINT('Origin',(10.4,4.,3.3));
#7136=CARTESIAN_POINT('',(10.5,4.,4.35));
#7137=CARTESIAN_POINT('Origin',(10.5,4.,3.3));
#7138=CARTESIAN_POINT('',(19.5,4.,4.35));
#7139=CARTESIAN_POINT('',(10.4,4.,4.35));
#7140=CARTESIAN_POINT('Origin',(19.5,4.,3.3));
#7141=CARTESIAN_POINT('Origin',(19.5,6.,1.6));
#7142=CARTESIAN_POINT('',(19.5,6.,1.6));
#7143=CARTESIAN_POINT('',(10.5,6.,1.6));
#7144=CARTESIAN_POINT('',(19.5,6.,1.6));
#7145=CARTESIAN_POINT('',(10.5,6.,5.8));
#7146=CARTESIAN_POINT('',(10.5,6.,1.6));
#7147=CARTESIAN_POINT('',(19.5,6.,5.8));
#7148=CARTESIAN_POINT('',(19.5,6.,5.8));
#7149=CARTESIAN_POINT('',(19.5,6.,1.6));
#7150=CARTESIAN_POINT('Origin',(19.5,-6.,1.6));
#7151=CARTESIAN_POINT('',(19.5,-6.,1.6));
#7152=CARTESIAN_POINT('',(19.5,-6.,1.6));
#7153=CARTESIAN_POINT('',(19.5,-6.,5.8));
#7154=CARTESIAN_POINT('',(19.5,-6.,5.8));
#7155=CARTESIAN_POINT('',(19.5,-6.,1.6));
#7156=CARTESIAN_POINT('Origin',(10.5,-6.,1.6));
#7157=CARTESIAN_POINT('',(10.5,-6.,1.6));
#7158=CARTESIAN_POINT('',(10.5,-6.,1.6));
#7159=CARTESIAN_POINT('',(10.5,-6.,5.8));
#7160=CARTESIAN_POINT('',(10.5,-6.,5.8));
#7161=CARTESIAN_POINT('',(10.5,-6.,1.6));
#7162=CARTESIAN_POINT('Origin',(10.5,6.,1.6));
#7163=CARTESIAN_POINT('',(10.5,6.,1.6));
#7164=CARTESIAN_POINT('',(10.5,6.,5.8));
#7165=CARTESIAN_POINT('Origin',(15.,0.,5.8));
#7166=CARTESIAN_POINT('Origin',(15.,0.,1.6));
#7795=UNCERTAINTY_MEASURE_WITH_UNIT(LENGTH_MEASURE(0.001),#7836,
'DISTANCE_ACCURACY_VALUE',
'Maximum model space distance between geometric entities at asserted c
onnectivities');
#7809=UNCERTAINTY_MEASURE_WITH_UNIT(LENGTH_MEASURE(0.001),#7836,
'DISTANCE_ACCURACY_VALUE',
'Maximum model space distance between geometric entities at asserted c
onnectivities');
#7821=(
GEOMETRIC_REPRESENTATION_CONTEXT(3)
GLOBAL_UNCERTAINTY_ASSIGNED_CONTEXT((#7795))
GLOBAL_UNIT_ASSIGNED_CONTEXT((#7836,#7838,#7839))
REPRESENTATION_CONTEXT('','3D')
);
#7835=(
GEOMETRIC_REPRESENTATION_CONTEXT(3)
GLOBAL_UNCERTAINTY_ASSIGNED_CONTEXT((#7809))
GLOBAL_UNIT_ASSIGNED_CONTEXT((#7836,#7838,#7839))
REPRESENTATION_CONTEXT('','3D')
);
#7836=(
LENGTH_UNIT()
NAMED_UNIT(*)
SI_UNIT(.CENTI.,.METRE.)
);
#7838=(
NAMED_UNIT(*)
PLANE_ANGLE_UNIT()
SI_UNIT($,.RADIAN.)
);
#7839=(
NAMED_UNIT(*)
SI_UNIT($,.STERADIAN.)
SOLID_ANGLE_UNIT()
);
#7851=SHAPE_DEFINITION_REPRESENTATION(#7876,#7957);
#7876=PRODUCT_DEFINITION_SHAPE('',$,#7983);
#7957=SHAPE_REPRESENTATION('',(#4823),#7821);
#7971=PRODUCT_DEFINITION_CONTEXT('part definition',#8048,'design');
#7983=PRODUCT_DEFINITION('Bushing housing','Bushing housing',#8008,#7971);
#8008=PRODUCT_DEFINITION_FORMATION('',$,#8061);
#8048=APPLICATION_CONTEXT(
'Core Data for Automotive Mechanical Design Process');
#8049=PRODUCT_CONTEXT('part definition',#8048,'mechanical');
#8061=PRODUCT('Bushing housing','Bushing housing','Bushing housing',(#8049));
#8117=COLOUR_RGB('Dark Blue',0.08,0.2,0.34);
#8118=FILL_AREA_STYLE_COLOUR('',#8117);
#8119=FILL_AREA_STYLE('',(#8118));
#8120=SURFACE_STYLE_FILL_AREA(#8119);
#8121=SURFACE_SIDE_STYLE('',(#8120));
#8122=SURFACE_STYLE_USAGE(.BOTH.,#8121);
#8123=PRESENTATION_STYLE_ASSIGNMENT((#8122));
ENDSEC;
END-ISO-10303-21;
